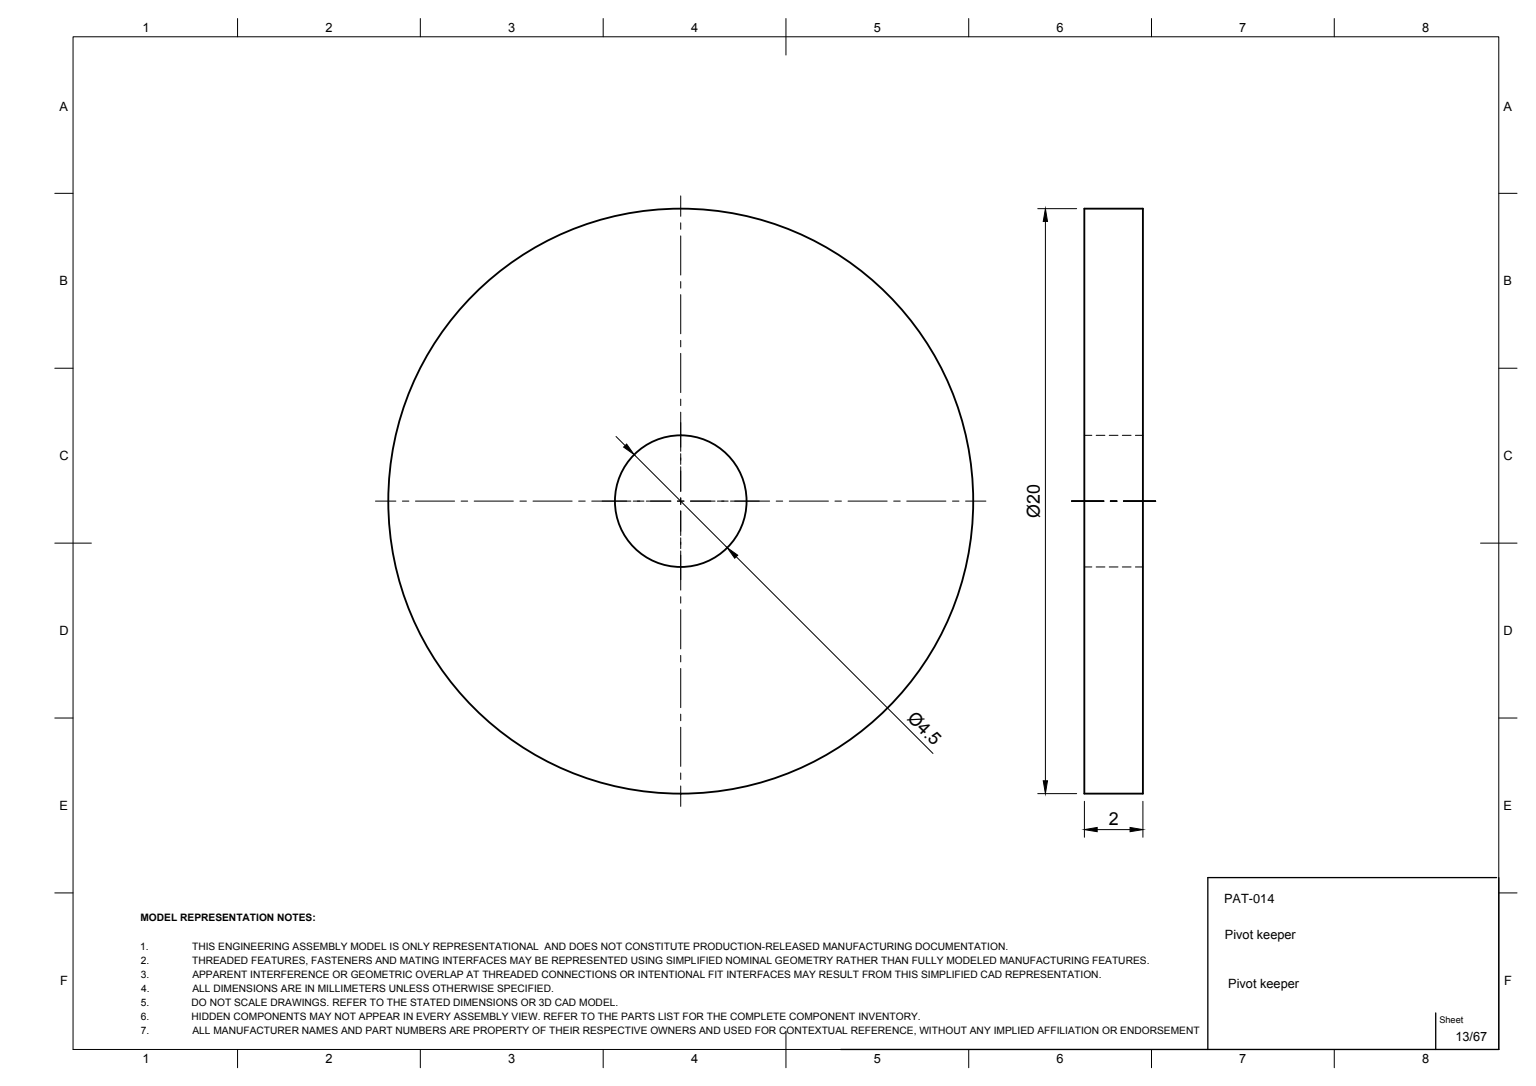
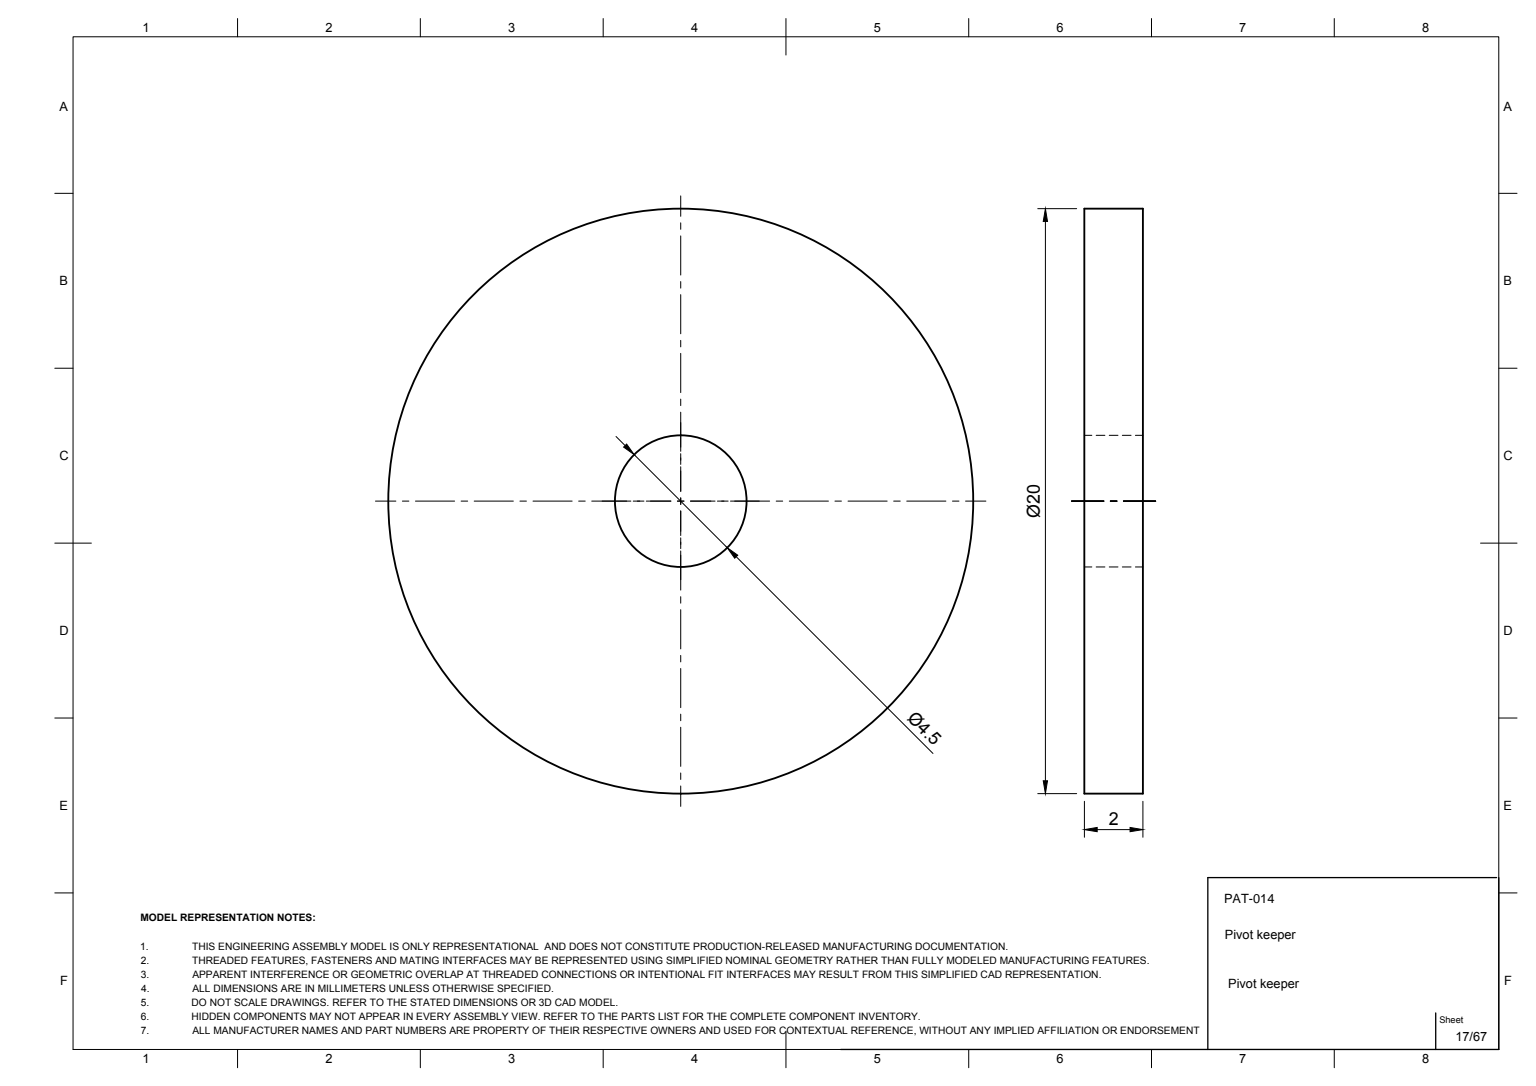
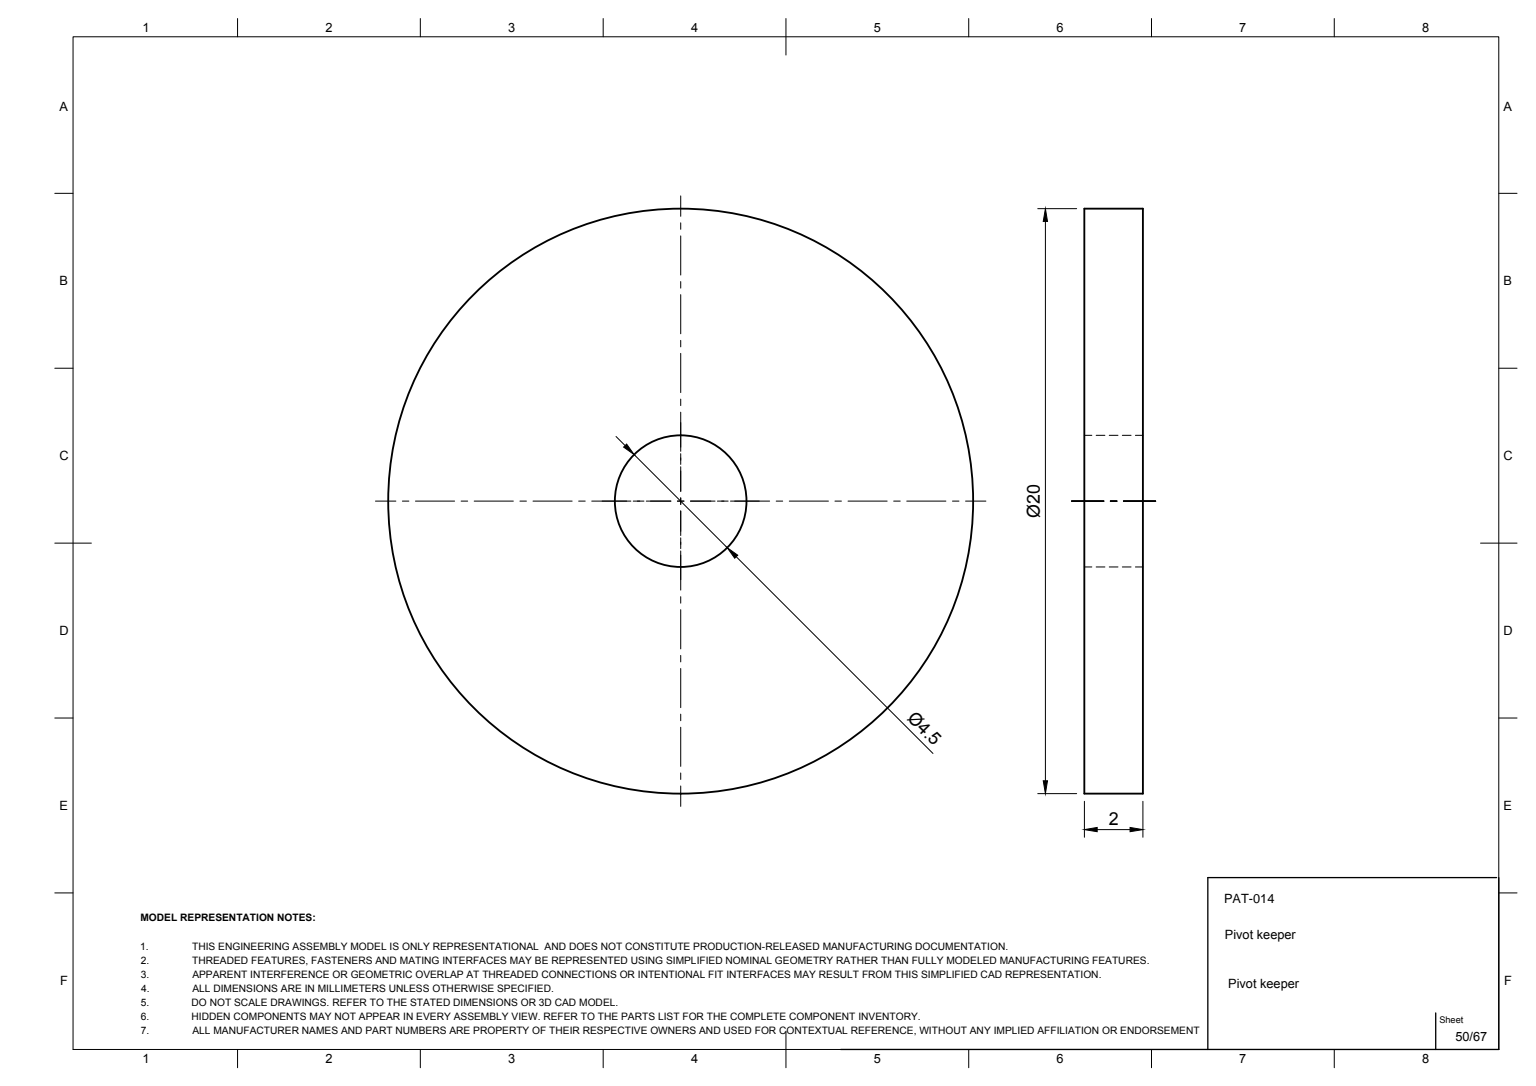
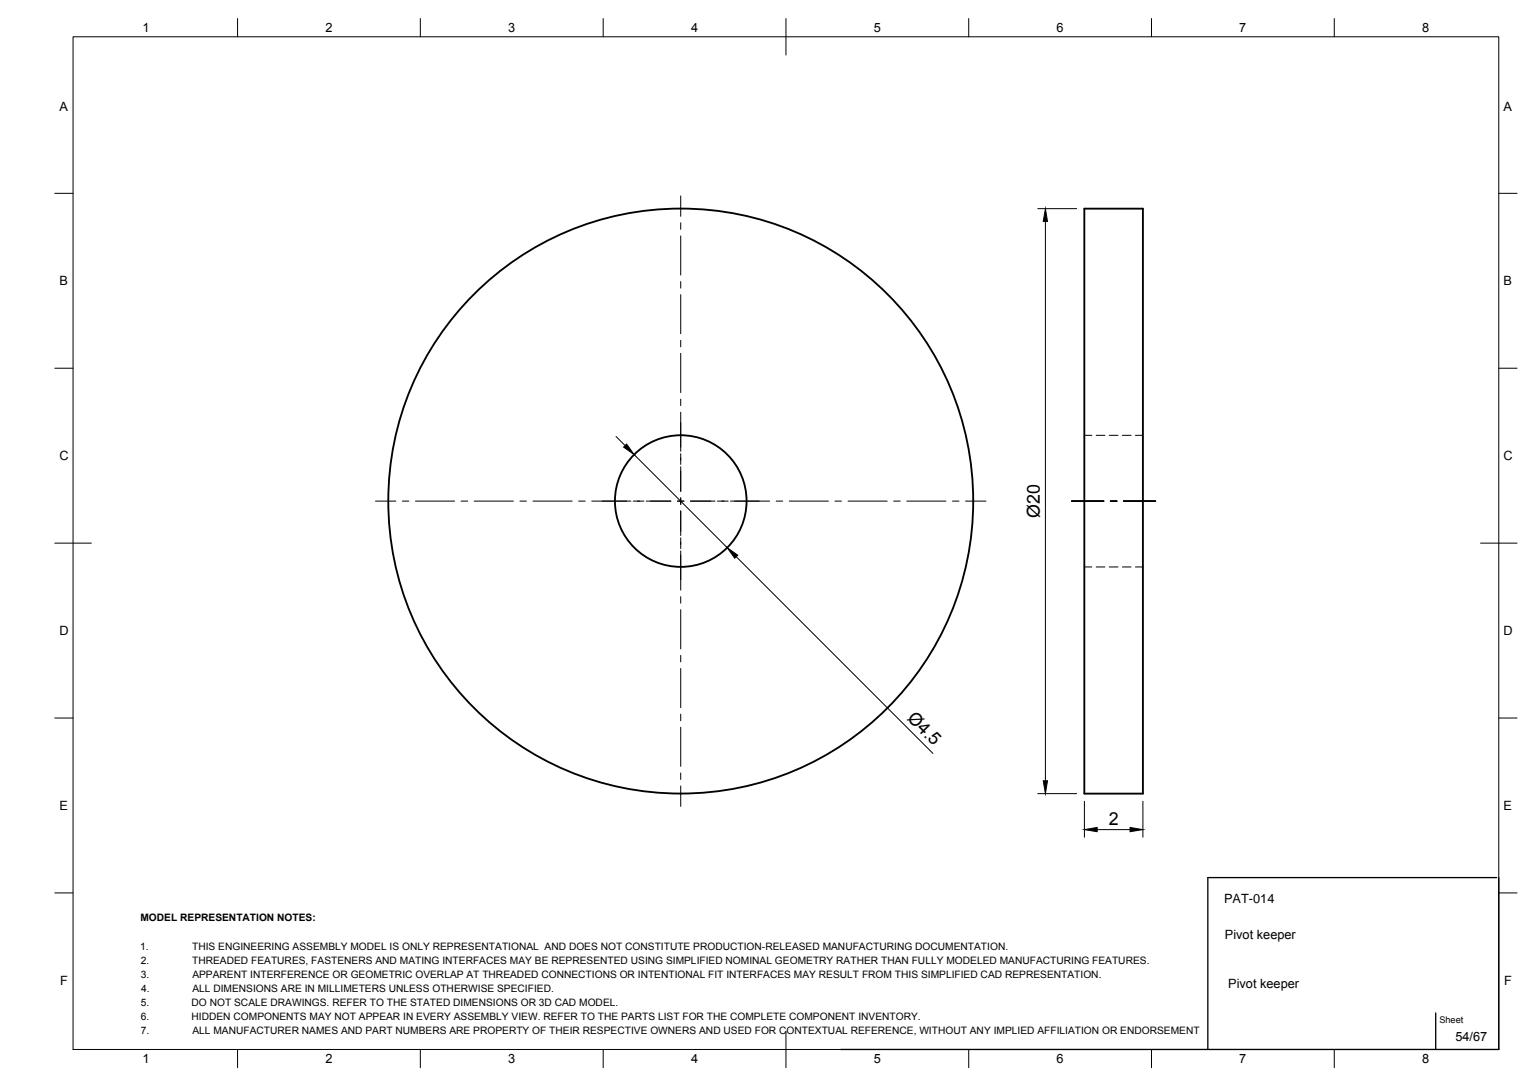
ISO-10303-21;
HEADER;
/* Generated by software containing ST-Developer
 * from STEP Tools, Inc. (www.steptools.com) 
 */

FILE_DESCRIPTION(
/* description */ ('Bin tilter linkage'),
/* implementation_level */ '2;1');

FILE_NAME(
/* name */ 'Pivot keeper.step',
/* time_stamp */ '2026-10-28T03:26:24-07:00',
/* author */ (''),
/* organization */ (''),
/* preprocessor_version */ 'ST-DEVELOPER v20.2',
/* originating_system */ 'Autodesk Translation Framework v15.17.0.0',
/* authorisation */ '');

FILE_SCHEMA (('AUTOMOTIVE_DESIGN { 1 0 10303 214 3 1 1 }'));
ENDSEC;

DATA;
#10=MECHANICAL_DESIGN_GEOMETRIC_PRESENTATION_REPRESENTATION('',(#870),#23728);
#658=SHAPE_REPRESENTATION_RELATIONSHIP('SRR','None',#24122,#764);
#764=ADVANCED_BREP_SHAPE_REPRESENTATION('',(#984),#23622);
#870=STYLED_ITEM('',(#24779),#984);
#984=MANIFOLD_SOLID_BREP('Body1',#12400);
#1156=FACE_BOUND('',#2825,.T.);
#1157=FACE_BOUND('',#2827,.T.);
#1539=PLANE('',#13857);
#1540=PLANE('',#13858);
#1976=FACE_OUTER_BOUND('',#2822,.T.);
#1977=FACE_OUTER_BOUND('',#2823,.T.);
#1978=FACE_OUTER_BOUND('',#2824,.T.);
#1979=FACE_OUTER_BOUND('',#2826,.T.);
#2822=EDGE_LOOP('',(#8775,#8776,#8777,#8778));
#2823=EDGE_LOOP('',(#8779,#8780,#8781,#8782));
#2824=EDGE_LOOP('',(#8783));
#2825=EDGE_LOOP('',(#8784));
#2826=EDGE_LOOP('',(#8785));
#2827=EDGE_LOOP('',(#8786));
#3972=LINE('',#20181,#4647);
#3973=LINE('',#20187,#4648);
#4647=VECTOR('',#15951,0.225);
#4648=VECTOR('',#15958,1.);
#5277=CIRCLE('',#13852,0.225);
#5278=CIRCLE('',#13853,0.225);
#5279=CIRCLE('',#13855,1.);
#5280=CIRCLE('',#13856,1.);
#6091=VERTEX_POINT('',#20178);
#6092=VERTEX_POINT('',#20180);
#6093=VERTEX_POINT('',#20184);
#6094=VERTEX_POINT('',#20186);
#7127=EDGE_CURVE('',#6091,#6091,#5277,.T.);
#7128=EDGE_CURVE('',#6091,#6092,#3972,.T.);
#7129=EDGE_CURVE('',#6092,#6092,#5278,.T.);
#7130=EDGE_CURVE('',#6093,#6093,#5279,.T.);
#7131=EDGE_CURVE('',#6093,#6094,#3973,.T.);
#7132=EDGE_CURVE('',#6094,#6094,#5280,.T.);
#8775=ORIENTED_EDGE('',*,*,#7127,.F.);
#8776=ORIENTED_EDGE('',*,*,#7128,.T.);
#8777=ORIENTED_EDGE('',*,*,#7129,.T.);
#8778=ORIENTED_EDGE('',*,*,#7128,.F.);
#8779=ORIENTED_EDGE('',*,*,#7130,.F.);
#8780=ORIENTED_EDGE('',*,*,#7131,.T.);
#8781=ORIENTED_EDGE('',*,*,#7132,.T.);
#8782=ORIENTED_EDGE('',*,*,#7131,.F.);
#8783=ORIENTED_EDGE('',*,*,#7130,.T.);
#8784=ORIENTED_EDGE('',*,*,#7127,.T.);
#8785=ORIENTED_EDGE('',*,*,#7132,.F.);
#8786=ORIENTED_EDGE('',*,*,#7129,.F.);
#11306=CYLINDRICAL_SURFACE('',#13851,0.225);
#11307=CYLINDRICAL_SURFACE('',#13854,1.);
#11701=ADVANCED_FACE('',(#1976),#11306,.F.);
#11702=ADVANCED_FACE('',(#1977),#11307,.T.);
#11703=ADVANCED_FACE('',(#1978,#1156),#1539,.T.);
#11704=ADVANCED_FACE('',(#1979,#1157),#1540,.F.);
#12400=CLOSED_SHELL('',(#11701,#11702,#11703,#11704));
#13850=AXIS2_PLACEMENT_3D('',#20176,#15945,#15946);
#13851=AXIS2_PLACEMENT_3D('',#20177,#15947,#15948);
#13852=AXIS2_PLACEMENT_3D('',#20179,#15949,#15950);
#13853=AXIS2_PLACEMENT_3D('',#20182,#15952,#15953);
#13854=AXIS2_PLACEMENT_3D('',#20183,#15954,#15955);
#13855=AXIS2_PLACEMENT_3D('',#20185,#15956,#15957);
#13856=AXIS2_PLACEMENT_3D('',#20188,#15959,#15960);
#13857=AXIS2_PLACEMENT_3D('',#20189,#15961,#15962);
#13858=AXIS2_PLACEMENT_3D('',#20190,#15963,#15964);
#15945=DIRECTION('axis',(0.,0.,1.));
#15946=DIRECTION('refdir',(1.,0.,0.));
#15947=DIRECTION('center_axis',(0.,1.,0.));
#15948=DIRECTION('ref_axis',(1.,0.,0.));
#15949=DIRECTION('center_axis',(0.,-1.,0.));
#15950=DIRECTION('ref_axis',(1.,0.,0.));
#15951=DIRECTION('',(0.,-1.,0.));
#15952=DIRECTION('center_axis',(0.,-1.,0.));
#15953=DIRECTION('ref_axis',(1.,0.,0.));
#15954=DIRECTION('center_axis',(0.,1.,0.));
#15955=DIRECTION('ref_axis',(1.,0.,0.));
#15956=DIRECTION('center_axis',(0.,1.,0.));
#15957=DIRECTION('ref_axis',(1.,0.,0.));
#15958=DIRECTION('',(0.,-1.,0.));
#15959=DIRECTION('center_axis',(0.,1.,0.));
#15960=DIRECTION('ref_axis',(1.,0.,0.));
#15961=DIRECTION('center_axis',(0.,1.,0.));
#15962=DIRECTION('ref_axis',(1.,0.,0.));
#15963=DIRECTION('center_axis',(0.,1.,0.));
#15964=DIRECTION('ref_axis',(1.,0.,0.));
#20176=CARTESIAN_POINT('',(0.,0.,0.));
#20177=CARTESIAN_POINT('Origin',(0.,-1.2,15.));
#20178=CARTESIAN_POINT('',(-0.225,-1.,15.));
#20179=CARTESIAN_POINT('Origin',(0.,-1.,15.));
#20180=CARTESIAN_POINT('',(-0.225,-1.2,15.));
#20181=CARTESIAN_POINT('',(-0.225,-1.2,15.));
#20182=CARTESIAN_POINT('Origin',(0.,-1.2,15.));
#20183=CARTESIAN_POINT('Origin',(0.,-1.2,15.));
#20184=CARTESIAN_POINT('',(-1.,-1.,15.));
#20185=CARTESIAN_POINT('Origin',(0.,-1.,15.));
#20186=CARTESIAN_POINT('',(-1.,-1.2,15.));
#20187=CARTESIAN_POINT('',(-1.,-1.2,15.));
#20188=CARTESIAN_POINT('Origin',(0.,-1.2,15.));
#20189=CARTESIAN_POINT('Origin',(0.,-1.,15.));
#20190=CARTESIAN_POINT('Origin',(0.,-1.2,15.));
#23505=UNCERTAINTY_MEASURE_WITH_UNIT(LENGTH_MEASURE(0.001),#23729,
'DISTANCE_ACCURACY_VALUE',
'Maximum model space distance between geometric entities at asserted c
onnectivities');
#23611=UNCERTAINTY_MEASURE_WITH_UNIT(LENGTH_MEASURE(0.001),#23729,
'DISTANCE_ACCURACY_VALUE',
'Maximum model space distance between geometric entities at asserted c
onnectivities');
#23622=(
GEOMETRIC_REPRESENTATION_CONTEXT(3)
GLOBAL_UNCERTAINTY_ASSIGNED_CONTEXT((#23505))
GLOBAL_UNIT_ASSIGNED_CONTEXT((#23729,#23731,#23732))
REPRESENTATION_CONTEXT('','3D')
);
#23728=(
GEOMETRIC_REPRESENTATION_CONTEXT(3)
GLOBAL_UNCERTAINTY_ASSIGNED_CONTEXT((#23611))
GLOBAL_UNIT_ASSIGNED_CONTEXT((#23729,#23731,#23732))
REPRESENTATION_CONTEXT('','3D')
);
#23729=(
LENGTH_UNIT()
NAMED_UNIT(*)
SI_UNIT(.CENTI.,.METRE.)
);
#23731=(
NAMED_UNIT(*)
PLANE_ANGLE_UNIT()
SI_UNIT($,.RADIAN.)
);
#23732=(
NAMED_UNIT(*)
SI_UNIT($,.STERADIAN.)
SOLID_ANGLE_UNIT()
);
#23743=SHAPE_DEFINITION_REPRESENTATION(#23859,#24122);
#23859=PRODUCT_DEFINITION_SHAPE('',$,#24239);
#24122=SHAPE_REPRESENTATION('',(#13850),#23622);
#24228=PRODUCT_DEFINITION_CONTEXT('part definition',#24578,'design');
#24239=PRODUCT_DEFINITION('Pivot keeper','Pivot keeper',#24355,#24228);
#24355=PRODUCT_DEFINITION_FORMATION('',$,#24590);
#24578=APPLICATION_CONTEXT(
'Core Data for Automotive Mechanical Design Process');
#24579=PRODUCT_CONTEXT('part definition',#24578,'mechanical');
#24590=PRODUCT('Pivot keeper','Pivot keeper','Pivot keeper',(#24579));
#24773=COLOUR_RGB('Off White',0.89,0.88,0.83);
#24774=FILL_AREA_STYLE_COLOUR('',#24773);
#24775=FILL_AREA_STYLE('',(#24774));
#24776=SURFACE_STYLE_FILL_AREA(#24775);
#24777=SURFACE_SIDE_STYLE('',(#24776));
#24778=SURFACE_STYLE_USAGE(.BOTH.,#24777);
#24779=PRESENTATION_STYLE_ASSIGNMENT((#24778));
ENDSEC;
END-ISO-10303-21;
